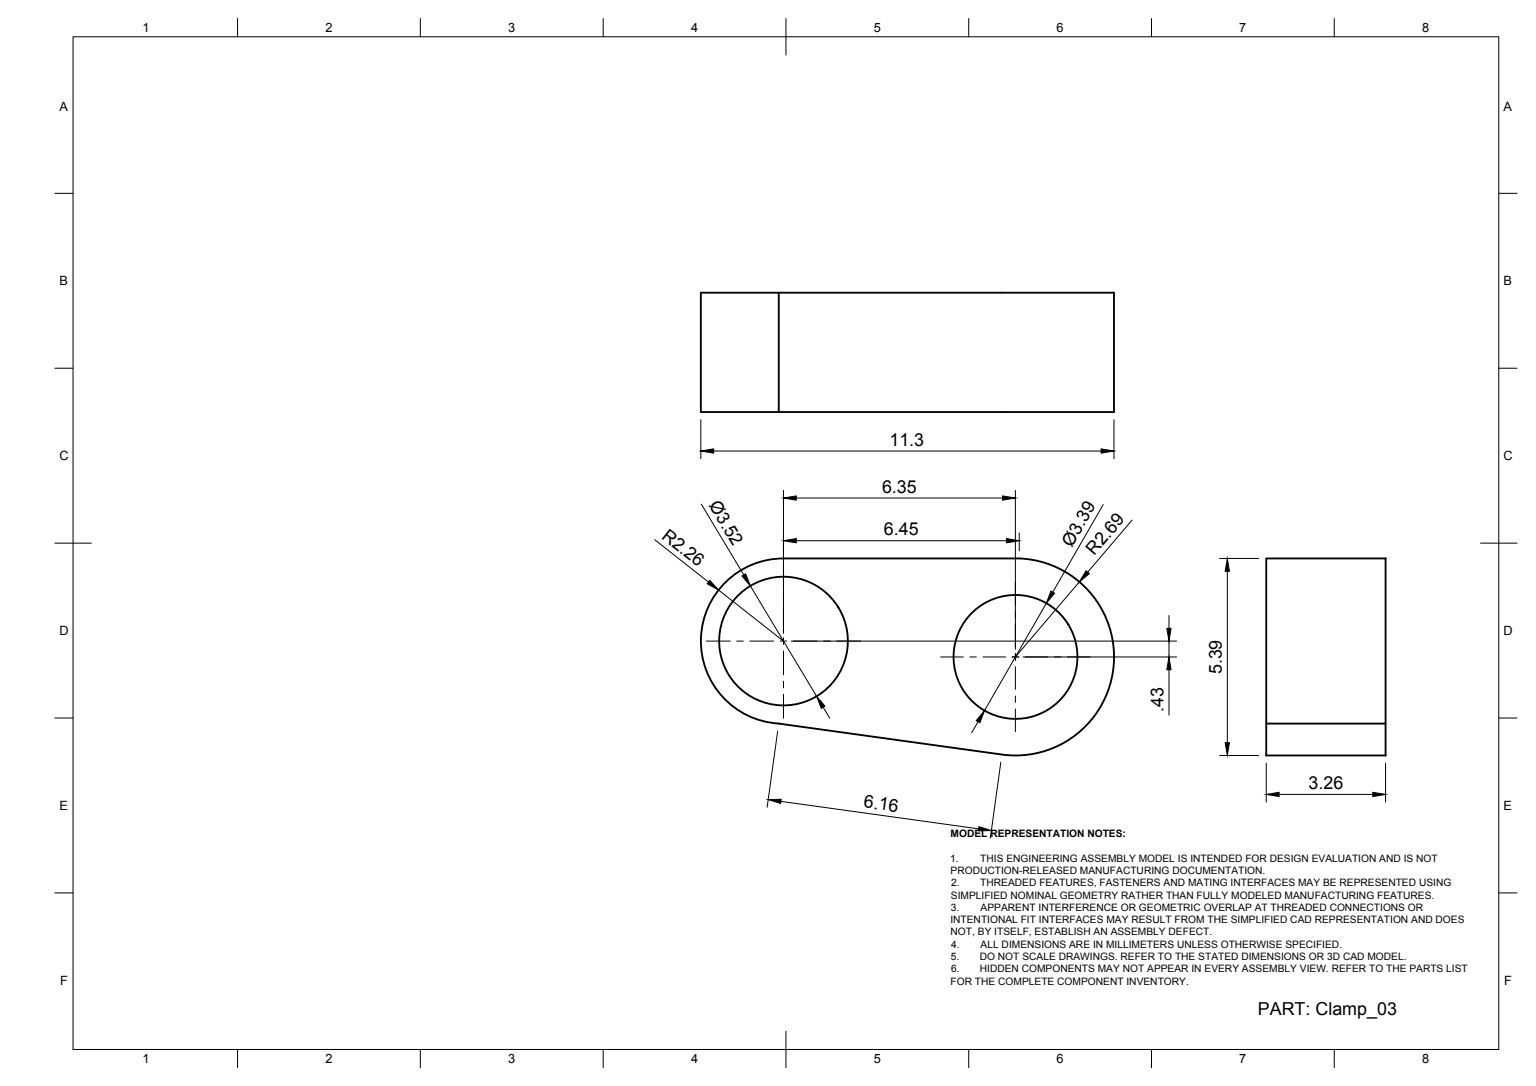
ISO-10303-21;
HEADER;
/* Generated by software containing ST-Developer
 * from STEP Tools, Inc. (www.steptools.com) 
 */

FILE_DESCRIPTION(
/* description */ (''),
/* implementation_level */ '2;1');

FILE_NAME(
/* name */ 'Clamp_03.step',
/* time_stamp */ '2026-10-05T16:20:14-07:00',
/* author */ (''),
/* organization */ (''),
/* preprocessor_version */ 'ST-DEVELOPER v20.2',
/* originating_system */ 'Autodesk Translation Framework v15.15.0.0',
/* authorisation */ '');

FILE_SCHEMA (('AUTOMOTIVE_DESIGN { 1 0 10303 214 3 1 1 }'));
ENDSEC;

DATA;
#10=MECHANICAL_DESIGN_GEOMETRIC_PRESENTATION_REPRESENTATION('',(#247),#23577);
#229=SHAPE_REPRESENTATION_RELATIONSHIP('SRR','None',#23612,#238);
#238=ADVANCED_BREP_SHAPE_REPRESENTATION('',(#256),#23568);
#247=STYLED_ITEM('',(#23666),#256);
#256=MANIFOLD_SOLID_BREP('Body1',#4157);
#265=FACE_BOUND('',#629,.T.);
#266=FACE_BOUND('',#630,.T.);
#267=FACE_BOUND('',#632,.T.);
#268=FACE_BOUND('',#633,.T.);
#300=PLANE('',#4277);
#301=PLANE('',#4281);
#302=PLANE('',#4282);
#303=PLANE('',#4283);
#396=FACE_OUTER_BOUND('',#622,.T.);
#397=FACE_OUTER_BOUND('',#623,.T.);
#398=FACE_OUTER_BOUND('',#624,.T.);
#399=FACE_OUTER_BOUND('',#625,.T.);
#400=FACE_OUTER_BOUND('',#626,.T.);
#401=FACE_OUTER_BOUND('',#627,.T.);
#402=FACE_OUTER_BOUND('',#628,.T.);
#403=FACE_OUTER_BOUND('',#631,.T.);
#622=EDGE_LOOP('',(#2637,#2638,#2639,#2640));
#623=EDGE_LOOP('',(#2641,#2642,#2643,#2644));
#624=EDGE_LOOP('',(#2645,#2646,#2647,#2648));
#625=EDGE_LOOP('',(#2649,#2650,#2651,#2652));
#626=EDGE_LOOP('',(#2653,#2654,#2655,#2656));
#627=EDGE_LOOP('',(#2657,#2658,#2659,#2660));
#628=EDGE_LOOP('',(#2661,#2662,#2663,#2664));
#629=EDGE_LOOP('',(#2665));
#630=EDGE_LOOP('',(#2666));
#631=EDGE_LOOP('',(#2667,#2668,#2669,#2670));
#632=EDGE_LOOP('',(#2671));
#633=EDGE_LOOP('',(#2672));
#883=LINE('',#5781,#1168);
#884=LINE('',#5787,#1169);
#885=LINE('',#5794,#1170);
#886=LINE('',#5797,#1171);
#887=LINE('',#5800,#1172);
#888=LINE('',#5802,#1173);
#889=LINE('',#5803,#1174);
#890=LINE('',#5809,#1175);
#891=LINE('',#5811,#1176);
#892=LINE('',#5812,#1177);
#1168=VECTOR('',#4682,1.75974879114541);
#1169=VECTOR('',#4689,1.69478250292167);
#1170=VECTOR('',#4696,10.);
#1171=VECTOR('',#4699,10.);
#1172=VECTOR('',#4702,10.);
#1173=VECTOR('',#4703,10.);
#1174=VECTOR('',#4704,10.);
#1175=VECTOR('',#4711,10.);
#1176=VECTOR('',#4714,10.);
#1177=VECTOR('',#4715,10.);
#1453=CIRCLE('',#4269,1.75974879114541);
#1454=CIRCLE('',#4270,1.75974879114541);
#1455=CIRCLE('',#4272,1.69478250292167);
#1456=CIRCLE('',#4273,1.69478250292167);
#1457=CIRCLE('',#4275,2.25974879114541);
#1458=CIRCLE('',#4276,2.25974879114541);
#1459=CIRCLE('',#4279,2.69478250292167);
#1460=CIRCLE('',#4280,2.69478250292167);
#1628=VERTEX_POINT('',#5778);
#1629=VERTEX_POINT('',#5780);
#1630=VERTEX_POINT('',#5784);
#1631=VERTEX_POINT('',#5786);
#1632=VERTEX_POINT('',#5790);
#1633=VERTEX_POINT('',#5791);
#1634=VERTEX_POINT('',#5793);
#1635=VERTEX_POINT('',#5795);
#1636=VERTEX_POINT('',#5799);
#1637=VERTEX_POINT('',#5801);
#1638=VERTEX_POINT('',#5805);
#1639=VERTEX_POINT('',#5807);
#2035=EDGE_CURVE('',#1628,#1628,#1453,.T.);
#2036=EDGE_CURVE('',#1628,#1629,#883,.T.);
#2037=EDGE_CURVE('',#1629,#1629,#1454,.T.);
#2038=EDGE_CURVE('',#1630,#1630,#1455,.T.);
#2039=EDGE_CURVE('',#1630,#1631,#884,.T.);
#2040=EDGE_CURVE('',#1631,#1631,#1456,.T.);
#2041=EDGE_CURVE('',#1632,#1633,#1457,.T.);
#2042=EDGE_CURVE('',#1633,#1634,#885,.T.);
#2043=EDGE_CURVE('',#1635,#1634,#1458,.T.);
#2044=EDGE_CURVE('',#1632,#1635,#886,.T.);
#2045=EDGE_CURVE('',#1636,#1632,#887,.T.);
#2046=EDGE_CURVE('',#1637,#1635,#888,.T.);
#2047=EDGE_CURVE('',#1636,#1637,#889,.T.);
#2048=EDGE_CURVE('',#1638,#1636,#1459,.T.);
#2049=EDGE_CURVE('',#1639,#1637,#1460,.T.);
#2050=EDGE_CURVE('',#1638,#1639,#890,.T.);
#2051=EDGE_CURVE('',#1633,#1638,#891,.T.);
#2052=EDGE_CURVE('',#1634,#1639,#892,.T.);
#2637=ORIENTED_EDGE('',*,*,#2035,.T.);
#2638=ORIENTED_EDGE('',*,*,#2036,.T.);
#2639=ORIENTED_EDGE('',*,*,#2037,.F.);
#2640=ORIENTED_EDGE('',*,*,#2036,.F.);
#2641=ORIENTED_EDGE('',*,*,#2038,.T.);
#2642=ORIENTED_EDGE('',*,*,#2039,.T.);
#2643=ORIENTED_EDGE('',*,*,#2040,.F.);
#2644=ORIENTED_EDGE('',*,*,#2039,.F.);
#2645=ORIENTED_EDGE('',*,*,#2041,.T.);
#2646=ORIENTED_EDGE('',*,*,#2042,.T.);
#2647=ORIENTED_EDGE('',*,*,#2043,.F.);
#2648=ORIENTED_EDGE('',*,*,#2044,.F.);
#2649=ORIENTED_EDGE('',*,*,#2045,.T.);
#2650=ORIENTED_EDGE('',*,*,#2044,.T.);
#2651=ORIENTED_EDGE('',*,*,#2046,.F.);
#2652=ORIENTED_EDGE('',*,*,#2047,.F.);
#2653=ORIENTED_EDGE('',*,*,#2048,.T.);
#2654=ORIENTED_EDGE('',*,*,#2047,.T.);
#2655=ORIENTED_EDGE('',*,*,#2049,.F.);
#2656=ORIENTED_EDGE('',*,*,#2050,.F.);
#2657=ORIENTED_EDGE('',*,*,#2051,.T.);
#2658=ORIENTED_EDGE('',*,*,#2050,.T.);
#2659=ORIENTED_EDGE('',*,*,#2052,.F.);
#2660=ORIENTED_EDGE('',*,*,#2042,.F.);
#2661=ORIENTED_EDGE('',*,*,#2052,.T.);
#2662=ORIENTED_EDGE('',*,*,#2049,.T.);
#2663=ORIENTED_EDGE('',*,*,#2046,.T.);
#2664=ORIENTED_EDGE('',*,*,#2043,.T.);
#2665=ORIENTED_EDGE('',*,*,#2040,.T.);
#2666=ORIENTED_EDGE('',*,*,#2037,.T.);
#2667=ORIENTED_EDGE('',*,*,#2051,.F.);
#2668=ORIENTED_EDGE('',*,*,#2041,.F.);
#2669=ORIENTED_EDGE('',*,*,#2045,.F.);
#2670=ORIENTED_EDGE('',*,*,#2048,.F.);
#2671=ORIENTED_EDGE('',*,*,#2038,.F.);
#2672=ORIENTED_EDGE('',*,*,#2035,.F.);
#3841=CYLINDRICAL_SURFACE('',#4268,1.75974879114541);
#3842=CYLINDRICAL_SURFACE('',#4271,1.69478250292167);
#3843=CYLINDRICAL_SURFACE('',#4274,2.25974879114541);
#3844=CYLINDRICAL_SURFACE('',#4278,2.69478250292167);
#3931=ADVANCED_FACE('',(#396),#3841,.F.);
#3932=ADVANCED_FACE('',(#397),#3842,.F.);
#3933=ADVANCED_FACE('',(#398),#3843,.T.);
#3934=ADVANCED_FACE('',(#399),#300,.T.);
#3935=ADVANCED_FACE('',(#400),#3844,.T.);
#3936=ADVANCED_FACE('',(#401),#301,.T.);
#3937=ADVANCED_FACE('',(#402,#265,#266),#302,.T.);
#3938=ADVANCED_FACE('',(#403,#267,#268),#303,.F.);
#4157=CLOSED_SHELL('',(#3931,#3932,#3933,#3934,#3935,#3936,#3937,#3938));
#4267=AXIS2_PLACEMENT_3D('',#5776,#4676,#4677);
#4268=AXIS2_PLACEMENT_3D('',#5777,#4678,#4679);
#4269=AXIS2_PLACEMENT_3D('',#5779,#4680,#4681);
#4270=AXIS2_PLACEMENT_3D('',#5782,#4683,#4684);
#4271=AXIS2_PLACEMENT_3D('',#5783,#4685,#4686);
#4272=AXIS2_PLACEMENT_3D('',#5785,#4687,#4688);
#4273=AXIS2_PLACEMENT_3D('',#5788,#4690,#4691);
#4274=AXIS2_PLACEMENT_3D('',#5789,#4692,#4693);
#4275=AXIS2_PLACEMENT_3D('',#5792,#4694,#4695);
#4276=AXIS2_PLACEMENT_3D('',#5796,#4697,#4698);
#4277=AXIS2_PLACEMENT_3D('',#5798,#4700,#4701);
#4278=AXIS2_PLACEMENT_3D('',#5804,#4705,#4706);
#4279=AXIS2_PLACEMENT_3D('',#5806,#4707,#4708);
#4280=AXIS2_PLACEMENT_3D('',#5808,#4709,#4710);
#4281=AXIS2_PLACEMENT_3D('',#5810,#4712,#4713);
#4282=AXIS2_PLACEMENT_3D('',#5813,#4716,#4717);
#4283=AXIS2_PLACEMENT_3D('',#5814,#4718,#4719);
#4676=DIRECTION('axis',(0.,0.,1.));
#4677=DIRECTION('refdir',(1.,0.,0.));
#4678=DIRECTION('center_axis',(0.,-1.,0.));
#4679=DIRECTION('ref_axis',(1.,0.,0.));
#4680=DIRECTION('center_axis',(0.,1.,0.));
#4681=DIRECTION('ref_axis',(1.,0.,0.));
#4682=DIRECTION('',(0.,-1.,0.));
#4683=DIRECTION('center_axis',(0.,1.,0.));
#4684=DIRECTION('ref_axis',(1.,0.,0.));
#4685=DIRECTION('center_axis',(0.,-1.,0.));
#4686=DIRECTION('ref_axis',(1.,0.,0.));
#4687=DIRECTION('center_axis',(0.,1.,0.));
#4688=DIRECTION('ref_axis',(1.,0.,0.));
#4689=DIRECTION('',(0.,-1.,0.));
#4690=DIRECTION('center_axis',(0.,1.,0.));
#4691=DIRECTION('ref_axis',(1.,0.,0.));
#4692=DIRECTION('center_axis',(0.,-1.,0.));
#4693=DIRECTION('ref_axis',(1.,0.,0.));
#4694=DIRECTION('center_axis',(0.,-1.,0.));
#4695=DIRECTION('ref_axis',(1.,0.,0.));
#4696=DIRECTION('',(0.,-1.,0.));
#4697=DIRECTION('center_axis',(0.,-1.,0.));
#4698=DIRECTION('ref_axis',(1.,0.,0.));
#4699=DIRECTION('',(0.,-1.,0.));
#4700=DIRECTION('center_axis',(-0.519736754180336,0.,-0.854326463568869));
#4701=DIRECTION('ref_axis',(0.854326463568869,8.60567687699182E-17,-0.519736754180336));
#4702=DIRECTION('',(0.854326463568868,8.60567687699182E-17,-0.519736754180336));
#4703=DIRECTION('',(0.854326463568868,8.60567687699182E-17,-0.519736754180336));
#4704=DIRECTION('',(0.,-1.,0.));
#4705=DIRECTION('center_axis',(0.,-1.,0.));
#4706=DIRECTION('ref_axis',(-0.805071965104942,0.,0.593177149763936));
#4707=DIRECTION('center_axis',(0.,-1.,0.));
#4708=DIRECTION('ref_axis',(1.,0.,0.));
#4709=DIRECTION('center_axis',(0.,-1.,0.));
#4710=DIRECTION('ref_axis',(1.,0.,0.));
#4711=DIRECTION('',(0.,-1.,0.));
#4712=DIRECTION('center_axis',(0.632123897156508,0.,0.774867329704685));
#4713=DIRECTION('ref_axis',(-0.774867329704685,-9.00832757384467E-17,0.632123897156508));
#4714=DIRECTION('',(-0.774867329704685,-9.00832757384467E-17,0.632123897156508));
#4715=DIRECTION('',(-0.774867329704685,-9.00832757384467E-17,0.632123897156508));
#4716=DIRECTION('center_axis',(0.,-1.,0.));
#4717=DIRECTION('ref_axis',(1.,0.,0.));
#4718=DIRECTION('center_axis',(0.,-1.,0.));
#4719=DIRECTION('ref_axis',(1.,0.,0.));
#5776=CARTESIAN_POINT('',(0.,0.,0.));
#5777=CARTESIAN_POINT('Origin',(37.3390884548007,1.63165946910082,-0.451167579126729));
#5778=CARTESIAN_POINT('',(35.5793396636553,1.63165946910082,-0.45116757912673));
#5779=CARTESIAN_POINT('Origin',(37.3390884548007,1.63165946910082,-0.451167579126729));
#5780=CARTESIAN_POINT('',(35.5793396636553,-1.63134053089918,-0.451167579126729));
#5781=CARTESIAN_POINT('',(35.5793396636553,1.63165946910082,-0.451167579126729));
#5782=CARTESIAN_POINT('Origin',(37.3390884548007,-1.63134053089918,-0.451167579126729));
#5783=CARTESIAN_POINT('Origin',(32.143405418954,1.63165946910082,3.2164639050219));
#5784=CARTESIAN_POINT('',(30.4486229160323,1.63165946910082,3.2164639050219));
#5785=CARTESIAN_POINT('Origin',(32.143405418954,1.63165946910082,3.2164639050219));
#5786=CARTESIAN_POINT('',(30.4486229160323,-1.63134053089918,3.2164639050219));
#5787=CARTESIAN_POINT('',(30.4486229160323,1.63165946910082,3.2164639050219));
#5788=CARTESIAN_POINT('Origin',(32.143405418954,-1.63134053089918,3.2164639050219));
#5789=CARTESIAN_POINT('Origin',(37.3390884548007,1.63165946910082,-0.451167579126729));
#5790=CARTESIAN_POINT('',(36.1646139528278,1.63165946910082,-2.38173077242002));
#5791=CARTESIAN_POINT('',(38.6217323111757,1.63165946910082,1.40928648824138));
#5792=CARTESIAN_POINT('Origin',(37.3390884548007,1.63165946910082,-0.451167579126729));
#5793=CARTESIAN_POINT('',(38.6217323111757,-1.63134053089918,1.40928648824138));
#5794=CARTESIAN_POINT('',(38.6217323111757,1.63165946910082,1.40928648824138));
#5795=CARTESIAN_POINT('',(36.1646139528278,-1.63134053089918,-2.38173077242002));
#5796=CARTESIAN_POINT('Origin',(37.3390884548007,-1.63134053089918,-0.451167579126729));
#5797=CARTESIAN_POINT('',(36.1646139528278,1.63165946910082,-2.38173077242002));
#5798=CARTESIAN_POINT('Origin',(30.6537580146004,1.63165946910082,0.970845204361578));
#5799=CARTESIAN_POINT('',(30.6537580146004,1.63165946910082,0.970845204361578));
#5800=CARTESIAN_POINT('',(30.6537580146004,1.63165946910082,0.970845204361578));
#5801=CARTESIAN_POINT('',(30.6537580146004,-1.63134053089918,0.970845204361578));
#5802=CARTESIAN_POINT('',(30.6537580146004,-1.63134053089918,0.970845204361578));
#5803=CARTESIAN_POINT('',(30.6537580146004,1.63165946910082,0.970845204361578));
#5804=CARTESIAN_POINT('Origin',(32.143405418954,1.63165946910082,3.2164639050219));
#5805=CARTESIAN_POINT('',(33.84684183669,1.63165946910082,5.30456282719571));
#5806=CARTESIAN_POINT('Origin',(32.143405418954,1.63165946910082,3.2164639050219));
#5807=CARTESIAN_POINT('',(33.84684183669,-1.63134053089918,5.30456282719571));
#5808=CARTESIAN_POINT('Origin',(32.143405418954,-1.63134053089918,3.2164639050219));
#5809=CARTESIAN_POINT('',(33.84684183669,1.63165946910082,5.30456282719571));
#5810=CARTESIAN_POINT('Origin',(38.6217323111757,1.63165946910082,1.40928648824138));
#5811=CARTESIAN_POINT('',(38.6217323111757,1.63165946910082,1.40928648824138));
#5812=CARTESIAN_POINT('',(38.6217323111757,-1.63134053089918,1.40928648824138));
#5813=CARTESIAN_POINT('Origin',(34.5237300809892,-1.63134053089918,1.60016501883572));
#5814=CARTESIAN_POINT('Origin',(34.5237300809892,1.63165946910082,1.60016501883572));
#23557=UNCERTAINTY_MEASURE_WITH_UNIT(LENGTH_MEASURE(0.01),#23578,
'DISTANCE_ACCURACY_VALUE',
'Maximum model space distance between geometric entities at asserted c
onnectivities');
#23566=UNCERTAINTY_MEASURE_WITH_UNIT(LENGTH_MEASURE(0.01),#23578,
'DISTANCE_ACCURACY_VALUE',
'Maximum model space distance between geometric entities at asserted c
onnectivities');
#23568=(
GEOMETRIC_REPRESENTATION_CONTEXT(3)
GLOBAL_UNCERTAINTY_ASSIGNED_CONTEXT((#23557))
GLOBAL_UNIT_ASSIGNED_CONTEXT((#23578,#23580,#23581))
REPRESENTATION_CONTEXT('','3D')
);
#23577=(
GEOMETRIC_REPRESENTATION_CONTEXT(3)
GLOBAL_UNCERTAINTY_ASSIGNED_CONTEXT((#23566))
GLOBAL_UNIT_ASSIGNED_CONTEXT((#23578,#23580,#23581))
REPRESENTATION_CONTEXT('','3D')
);
#23578=(
LENGTH_UNIT()
NAMED_UNIT(*)
SI_UNIT(.MILLI.,.METRE.)
);
#23580=(
NAMED_UNIT(*)
PLANE_ANGLE_UNIT()
SI_UNIT($,.RADIAN.)
);
#23581=(
NAMED_UNIT(*)
SI_UNIT($,.STERADIAN.)
SOLID_ANGLE_UNIT()
);
#23583=SHAPE_DEFINITION_REPRESENTATION(#23593,#23612);
#23593=PRODUCT_DEFINITION_SHAPE('',$,#23623);
#23612=SHAPE_REPRESENTATION('',(#4267),#23568);
#23621=PRODUCT_DEFINITION_CONTEXT('part definition',#23653,'design');
#23623=PRODUCT_DEFINITION('Clamp_03','Clamp_03',#23633,#23621);
#23633=PRODUCT_DEFINITION_FORMATION('',$,#23656);
#23653=APPLICATION_CONTEXT(
'Core Data for Automotive Mechanical Design Process');
#23654=PRODUCT_CONTEXT('part definition',#23653,'mechanical');
#23656=PRODUCT('Clamp_03','Clamp_03',$,(#23654));
#23666=PRESENTATION_STYLE_ASSIGNMENT((#23671));
#23671=SURFACE_STYLE_USAGE(.BOTH.,#23676);
#23676=SURFACE_SIDE_STYLE('',(#23681));
#23681=SURFACE_STYLE_FILL_AREA(#23686);
#23686=FILL_AREA_STYLE('Opaque(210,210,210)',(#23691));
#23691=FILL_AREA_STYLE_COLOUR('Opaque(210,210,210)',#23696);
#23696=COLOUR_RGB('Opaque(210,210,210)', 0.09019608, 0.27058824, 0.51372549);
ENDSEC;
END-ISO-10303-21;
